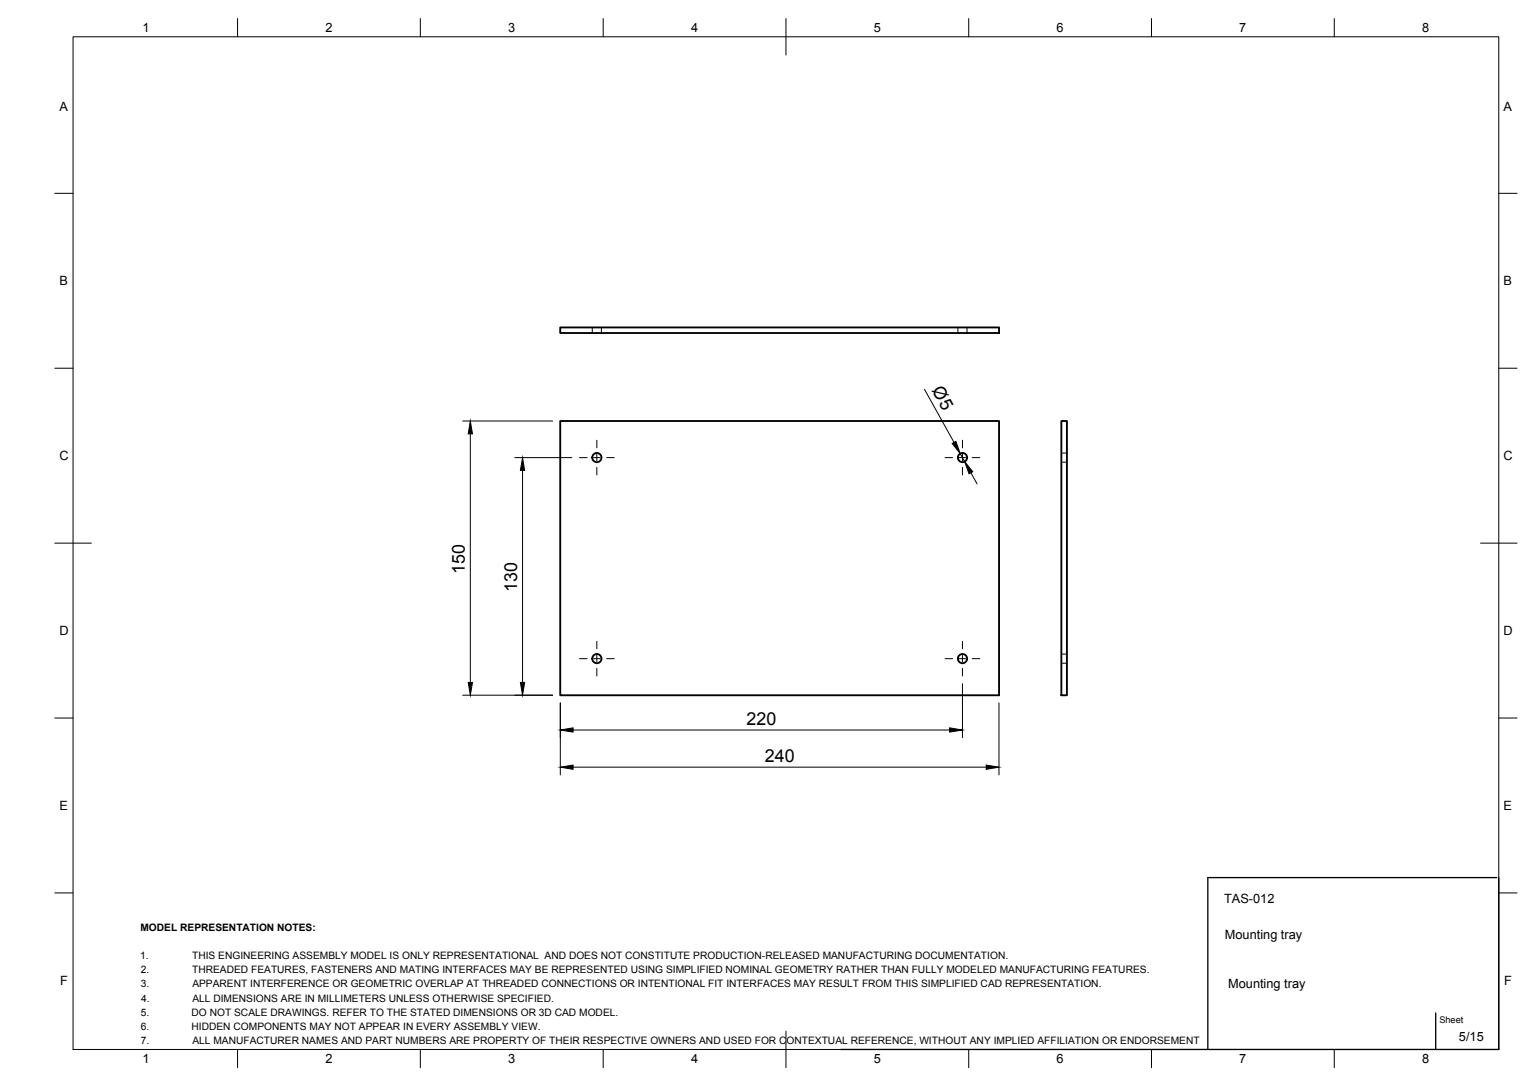
ISO-10303-21;
HEADER;
/* Generated by software containing ST-Developer
 * from STEP Tools, Inc. (www.steptools.com) 
 */

FILE_DESCRIPTION(
/* description */ (
'Independent welded steel electronics enclosure with removable sealed 
lid, internal mounting tray and two threaded cable entries. 300 x 220 
mm body. No ingress or electrical safety rating assigned.'),
/* implementation_level */ '2;1');

FILE_NAME(
/* name */ 'Mounting tray.step',
/* time_stamp */ '2026-11-14T09:13:27-08:00',
/* author */ (''),
/* organization */ (''),
/* preprocessor_version */ 'ST-DEVELOPER v20.2',
/* originating_system */ 'Autodesk Translation Framework v15.17.0.0',
/* authorisation */ '');

FILE_SCHEMA (('AUTOMOTIVE_DESIGN { 1 0 10303 214 3 1 1 }'));
ENDSEC;

DATA;
#10=MECHANICAL_DESIGN_GEOMETRIC_PRESENTATION_REPRESENTATION('',(#975),#94412);
#945=SHAPE_REPRESENTATION_RELATIONSHIP('SRR','None',#94497,#960);
#960=ADVANCED_BREP_SHAPE_REPRESENTATION('',(#990),#94406);
#975=STYLED_ITEM('',(#94580),#990);
#990=MANIFOLD_SOLID_BREP('Body1',#8260);
#1035=FACE_BOUND('',#1790,.T.);
#1036=FACE_BOUND('',#1791,.T.);
#1037=FACE_BOUND('',#1792,.T.);
#1038=FACE_BOUND('',#1793,.T.);
#1039=FACE_BOUND('',#1795,.T.);
#1040=FACE_BOUND('',#1796,.T.);
#1041=FACE_BOUND('',#1797,.T.);
#1042=FACE_BOUND('',#1798,.T.);
#1125=PLANE('',#8767);
#1126=PLANE('',#8768);
#1127=PLANE('',#8769);
#1128=PLANE('',#8770);
#1129=PLANE('',#8771);
#1130=PLANE('',#8772);
#1386=FACE_OUTER_BOUND('',#1781,.T.);
#1387=FACE_OUTER_BOUND('',#1782,.T.);
#1388=FACE_OUTER_BOUND('',#1783,.T.);
#1389=FACE_OUTER_BOUND('',#1784,.T.);
#1390=FACE_OUTER_BOUND('',#1785,.T.);
#1391=FACE_OUTER_BOUND('',#1786,.T.);
#1392=FACE_OUTER_BOUND('',#1787,.T.);
#1393=FACE_OUTER_BOUND('',#1788,.T.);
#1394=FACE_OUTER_BOUND('',#1789,.T.);
#1395=FACE_OUTER_BOUND('',#1794,.T.);
#1781=EDGE_LOOP('',(#6764,#6765,#6766,#6767));
#1782=EDGE_LOOP('',(#6768,#6769,#6770,#6771));
#1783=EDGE_LOOP('',(#6772,#6773,#6774,#6775));
#1784=EDGE_LOOP('',(#6776,#6777,#6778,#6779));
#1785=EDGE_LOOP('',(#6780,#6781,#6782,#6783));
#1786=EDGE_LOOP('',(#6784,#6785,#6786,#6787));
#1787=EDGE_LOOP('',(#6788,#6789,#6790,#6791));
#1788=EDGE_LOOP('',(#6792,#6793,#6794,#6795));
#1789=EDGE_LOOP('',(#6796,#6797,#6798,#6799));
#1790=EDGE_LOOP('',(#6800));
#1791=EDGE_LOOP('',(#6801));
#1792=EDGE_LOOP('',(#6802));
#1793=EDGE_LOOP('',(#6803));
#1794=EDGE_LOOP('',(#6804,#6805,#6806,#6807));
#1795=EDGE_LOOP('',(#6808));
#1796=EDGE_LOOP('',(#6809));
#1797=EDGE_LOOP('',(#6810));
#1798=EDGE_LOOP('',(#6811));
#2203=LINE('',#59828,#2601);
#2204=LINE('',#59834,#2602);
#2205=LINE('',#59840,#2603);
#2206=LINE('',#59846,#2604);
#2207=LINE('',#59851,#2605);
#2208=LINE('',#59853,#2606);
#2209=LINE('',#59855,#2607);
#2210=LINE('',#59856,#2608);
#2211=LINE('',#59859,#2609);
#2212=LINE('',#59861,#2610);
#2213=LINE('',#59862,#2611);
#2214=LINE('',#59865,#2612);
#2215=LINE('',#59867,#2613);
#2216=LINE('',#59868,#2614);
#2217=LINE('',#59870,#2615);
#2218=LINE('',#59871,#2616);
#2601=VECTOR('',#9863,2.5);
#2602=VECTOR('',#9870,2.5);
#2603=VECTOR('',#9877,2.5);
#2604=VECTOR('',#9884,2.5);
#2605=VECTOR('',#9889,10.);
#2606=VECTOR('',#9890,10.);
#2607=VECTOR('',#9891,10.);
#2608=VECTOR('',#9892,10.);
#2609=VECTOR('',#9895,10.);
#2610=VECTOR('',#9896,10.);
#2611=VECTOR('',#9897,10.);
#2612=VECTOR('',#9900,10.);
#2613=VECTOR('',#9901,10.);
#2614=VECTOR('',#9902,10.);
#2615=VECTOR('',#9905,10.);
#2616=VECTOR('',#9906,10.);
#2802=CIRCLE('',#8756,2.5);
#2803=CIRCLE('',#8757,2.5);
#2804=CIRCLE('',#8759,2.5);
#2805=CIRCLE('',#8760,2.5);
#2806=CIRCLE('',#8762,2.5);
#2807=CIRCLE('',#8763,2.5);
#2808=CIRCLE('',#8765,2.5);
#2809=CIRCLE('',#8766,2.5);
#3476=VERTEX_POINT('',#59825);
#3477=VERTEX_POINT('',#59827);
#3478=VERTEX_POINT('',#59831);
#3479=VERTEX_POINT('',#59833);
#3480=VERTEX_POINT('',#59837);
#3481=VERTEX_POINT('',#59839);
#3482=VERTEX_POINT('',#59843);
#3483=VERTEX_POINT('',#59845);
#3484=VERTEX_POINT('',#59849);
#3485=VERTEX_POINT('',#59850);
#3486=VERTEX_POINT('',#59852);
#3487=VERTEX_POINT('',#59854);
#3488=VERTEX_POINT('',#59858);
#3489=VERTEX_POINT('',#59860);
#3490=VERTEX_POINT('',#59864);
#3491=VERTEX_POINT('',#59866);
#4647=EDGE_CURVE('',#3476,#3476,#2802,.T.);
#4648=EDGE_CURVE('',#3476,#3477,#2203,.T.);
#4649=EDGE_CURVE('',#3477,#3477,#2803,.T.);
#4650=EDGE_CURVE('',#3478,#3478,#2804,.T.);
#4651=EDGE_CURVE('',#3478,#3479,#2204,.T.);
#4652=EDGE_CURVE('',#3479,#3479,#2805,.T.);
#4653=EDGE_CURVE('',#3480,#3480,#2806,.T.);
#4654=EDGE_CURVE('',#3480,#3481,#2205,.T.);
#4655=EDGE_CURVE('',#3481,#3481,#2807,.T.);
#4656=EDGE_CURVE('',#3482,#3482,#2808,.T.);
#4657=EDGE_CURVE('',#3482,#3483,#2206,.T.);
#4658=EDGE_CURVE('',#3483,#3483,#2809,.T.);
#4659=EDGE_CURVE('',#3484,#3485,#2207,.T.);
#4660=EDGE_CURVE('',#3485,#3486,#2208,.T.);
#4661=EDGE_CURVE('',#3487,#3486,#2209,.T.);
#4662=EDGE_CURVE('',#3484,#3487,#2210,.T.);
#4663=EDGE_CURVE('',#3488,#3484,#2211,.T.);
#4664=EDGE_CURVE('',#3489,#3487,#2212,.T.);
#4665=EDGE_CURVE('',#3488,#3489,#2213,.T.);
#4666=EDGE_CURVE('',#3490,#3488,#2214,.T.);
#4667=EDGE_CURVE('',#3491,#3489,#2215,.T.);
#4668=EDGE_CURVE('',#3490,#3491,#2216,.T.);
#4669=EDGE_CURVE('',#3485,#3490,#2217,.T.);
#4670=EDGE_CURVE('',#3486,#3491,#2218,.T.);
#6764=ORIENTED_EDGE('',*,*,#4647,.F.);
#6765=ORIENTED_EDGE('',*,*,#4648,.T.);
#6766=ORIENTED_EDGE('',*,*,#4649,.F.);
#6767=ORIENTED_EDGE('',*,*,#4648,.F.);
#6768=ORIENTED_EDGE('',*,*,#4650,.F.);
#6769=ORIENTED_EDGE('',*,*,#4651,.T.);
#6770=ORIENTED_EDGE('',*,*,#4652,.F.);
#6771=ORIENTED_EDGE('',*,*,#4651,.F.);
#6772=ORIENTED_EDGE('',*,*,#4653,.F.);
#6773=ORIENTED_EDGE('',*,*,#4654,.T.);
#6774=ORIENTED_EDGE('',*,*,#4655,.F.);
#6775=ORIENTED_EDGE('',*,*,#4654,.F.);
#6776=ORIENTED_EDGE('',*,*,#4656,.F.);
#6777=ORIENTED_EDGE('',*,*,#4657,.T.);
#6778=ORIENTED_EDGE('',*,*,#4658,.F.);
#6779=ORIENTED_EDGE('',*,*,#4657,.F.);
#6780=ORIENTED_EDGE('',*,*,#4659,.T.);
#6781=ORIENTED_EDGE('',*,*,#4660,.T.);
#6782=ORIENTED_EDGE('',*,*,#4661,.F.);
#6783=ORIENTED_EDGE('',*,*,#4662,.F.);
#6784=ORIENTED_EDGE('',*,*,#4663,.T.);
#6785=ORIENTED_EDGE('',*,*,#4662,.T.);
#6786=ORIENTED_EDGE('',*,*,#4664,.F.);
#6787=ORIENTED_EDGE('',*,*,#4665,.F.);
#6788=ORIENTED_EDGE('',*,*,#4666,.T.);
#6789=ORIENTED_EDGE('',*,*,#4665,.T.);
#6790=ORIENTED_EDGE('',*,*,#4667,.F.);
#6791=ORIENTED_EDGE('',*,*,#4668,.F.);
#6792=ORIENTED_EDGE('',*,*,#4669,.T.);
#6793=ORIENTED_EDGE('',*,*,#4668,.T.);
#6794=ORIENTED_EDGE('',*,*,#4670,.F.);
#6795=ORIENTED_EDGE('',*,*,#4660,.F.);
#6796=ORIENTED_EDGE('',*,*,#4670,.T.);
#6797=ORIENTED_EDGE('',*,*,#4667,.T.);
#6798=ORIENTED_EDGE('',*,*,#4664,.T.);
#6799=ORIENTED_EDGE('',*,*,#4661,.T.);
#6800=ORIENTED_EDGE('',*,*,#4647,.T.);
#6801=ORIENTED_EDGE('',*,*,#4650,.T.);
#6802=ORIENTED_EDGE('',*,*,#4653,.T.);
#6803=ORIENTED_EDGE('',*,*,#4656,.T.);
#6804=ORIENTED_EDGE('',*,*,#4669,.F.);
#6805=ORIENTED_EDGE('',*,*,#4659,.F.);
#6806=ORIENTED_EDGE('',*,*,#4663,.F.);
#6807=ORIENTED_EDGE('',*,*,#4666,.F.);
#6808=ORIENTED_EDGE('',*,*,#4649,.T.);
#6809=ORIENTED_EDGE('',*,*,#4652,.T.);
#6810=ORIENTED_EDGE('',*,*,#4655,.T.);
#6811=ORIENTED_EDGE('',*,*,#4658,.T.);
#7810=CYLINDRICAL_SURFACE('',#8755,2.5);
#7811=CYLINDRICAL_SURFACE('',#8758,2.5);
#7812=CYLINDRICAL_SURFACE('',#8761,2.5);
#7813=CYLINDRICAL_SURFACE('',#8764,2.5);
#8123=ADVANCED_FACE('',(#1386),#7810,.F.);
#8124=ADVANCED_FACE('',(#1387),#7811,.F.);
#8125=ADVANCED_FACE('',(#1388),#7812,.F.);
#8126=ADVANCED_FACE('',(#1389),#7813,.F.);
#8127=ADVANCED_FACE('',(#1390),#1125,.T.);
#8128=ADVANCED_FACE('',(#1391),#1126,.T.);
#8129=ADVANCED_FACE('',(#1392),#1127,.T.);
#8130=ADVANCED_FACE('',(#1393),#1128,.T.);
#8131=ADVANCED_FACE('',(#1394,#1035,#1036,#1037,#1038),#1129,.T.);
#8132=ADVANCED_FACE('',(#1395,#1039,#1040,#1041,#1042),#1130,.F.);
#8260=CLOSED_SHELL('',(#8123,#8124,#8125,#8126,#8127,#8128,#8129,#8130,
#8131,#8132));
#8754=AXIS2_PLACEMENT_3D('',#59823,#9857,#9858);
#8755=AXIS2_PLACEMENT_3D('',#59824,#9859,#9860);
#8756=AXIS2_PLACEMENT_3D('',#59826,#9861,#9862);
#8757=AXIS2_PLACEMENT_3D('',#59829,#9864,#9865);
#8758=AXIS2_PLACEMENT_3D('',#59830,#9866,#9867);
#8759=AXIS2_PLACEMENT_3D('',#59832,#9868,#9869);
#8760=AXIS2_PLACEMENT_3D('',#59835,#9871,#9872);
#8761=AXIS2_PLACEMENT_3D('',#59836,#9873,#9874);
#8762=AXIS2_PLACEMENT_3D('',#59838,#9875,#9876);
#8763=AXIS2_PLACEMENT_3D('',#59841,#9878,#9879);
#8764=AXIS2_PLACEMENT_3D('',#59842,#9880,#9881);
#8765=AXIS2_PLACEMENT_3D('',#59844,#9882,#9883);
#8766=AXIS2_PLACEMENT_3D('',#59847,#9885,#9886);
#8767=AXIS2_PLACEMENT_3D('',#59848,#9887,#9888);
#8768=AXIS2_PLACEMENT_3D('',#59857,#9893,#9894);
#8769=AXIS2_PLACEMENT_3D('',#59863,#9898,#9899);
#8770=AXIS2_PLACEMENT_3D('',#59869,#9903,#9904);
#8771=AXIS2_PLACEMENT_3D('',#59872,#9907,#9908);
#8772=AXIS2_PLACEMENT_3D('',#59873,#9909,#9910);
#9857=DIRECTION('axis',(0.,0.,1.));
#9858=DIRECTION('refdir',(1.,0.,0.));
#9859=DIRECTION('center_axis',(0.,0.,-1.));
#9860=DIRECTION('ref_axis',(1.,0.,0.));
#9861=DIRECTION('center_axis',(0.,0.,-1.));
#9862=DIRECTION('ref_axis',(1.,0.,0.));
#9863=DIRECTION('',(0.,0.,-1.));
#9864=DIRECTION('center_axis',(0.,0.,1.));
#9865=DIRECTION('ref_axis',(1.,0.,0.));
#9866=DIRECTION('center_axis',(0.,0.,-1.));
#9867=DIRECTION('ref_axis',(1.,0.,0.));
#9868=DIRECTION('center_axis',(0.,0.,-1.));
#9869=DIRECTION('ref_axis',(1.,0.,0.));
#9870=DIRECTION('',(0.,0.,-1.));
#9871=DIRECTION('center_axis',(0.,0.,1.));
#9872=DIRECTION('ref_axis',(1.,0.,0.));
#9873=DIRECTION('center_axis',(0.,0.,-1.));
#9874=DIRECTION('ref_axis',(1.,0.,0.));
#9875=DIRECTION('center_axis',(0.,0.,-1.));
#9876=DIRECTION('ref_axis',(1.,0.,0.));
#9877=DIRECTION('',(0.,0.,-1.));
#9878=DIRECTION('center_axis',(0.,0.,1.));
#9879=DIRECTION('ref_axis',(1.,0.,0.));
#9880=DIRECTION('center_axis',(0.,0.,-1.));
#9881=DIRECTION('ref_axis',(1.,0.,0.));
#9882=DIRECTION('center_axis',(0.,0.,-1.));
#9883=DIRECTION('ref_axis',(1.,0.,0.));
#9884=DIRECTION('',(0.,0.,-1.));
#9885=DIRECTION('center_axis',(0.,0.,1.));
#9886=DIRECTION('ref_axis',(1.,0.,0.));
#9887=DIRECTION('center_axis',(0.,1.,0.));
#9888=DIRECTION('ref_axis',(-1.,0.,0.));
#9889=DIRECTION('',(-1.,0.,0.));
#9890=DIRECTION('',(0.,0.,1.));
#9891=DIRECTION('',(-1.,0.,0.));
#9892=DIRECTION('',(0.,0.,1.));
#9893=DIRECTION('center_axis',(1.,0.,0.));
#9894=DIRECTION('ref_axis',(0.,1.,0.));
#9895=DIRECTION('',(0.,1.,0.));
#9896=DIRECTION('',(0.,1.,0.));
#9897=DIRECTION('',(0.,0.,1.));
#9898=DIRECTION('center_axis',(0.,-1.,0.));
#9899=DIRECTION('ref_axis',(1.,0.,0.));
#9900=DIRECTION('',(1.,0.,0.));
#9901=DIRECTION('',(1.,0.,0.));
#9902=DIRECTION('',(0.,0.,1.));
#9903=DIRECTION('center_axis',(-1.,0.,0.));
#9904=DIRECTION('ref_axis',(0.,-1.,0.));
#9905=DIRECTION('',(0.,-1.,0.));
#9906=DIRECTION('',(0.,-1.,0.));
#9907=DIRECTION('center_axis',(0.,0.,1.));
#9908=DIRECTION('ref_axis',(1.,0.,0.));
#9909=DIRECTION('center_axis',(0.,0.,1.));
#9910=DIRECTION('ref_axis',(1.,0.,0.));
#59823=CARTESIAN_POINT('',(0.,0.,0.));
#59824=CARTESIAN_POINT('Origin',(100.,-55.,1.5));
#59825=CARTESIAN_POINT('',(97.5,-55.,3.));
#59826=CARTESIAN_POINT('Origin',(100.,-55.,3.));
#59827=CARTESIAN_POINT('',(97.5,-55.,0.));
#59828=CARTESIAN_POINT('',(97.5,-55.,1.5));
#59829=CARTESIAN_POINT('Origin',(100.,-55.,0.));
#59830=CARTESIAN_POINT('Origin',(-100.,-55.,1.5));
#59831=CARTESIAN_POINT('',(-102.5,-55.,3.));
#59832=CARTESIAN_POINT('Origin',(-100.,-55.,3.));
#59833=CARTESIAN_POINT('',(-102.5,-55.,0.));
#59834=CARTESIAN_POINT('',(-102.5,-55.,1.5));
#59835=CARTESIAN_POINT('Origin',(-100.,-55.,0.));
#59836=CARTESIAN_POINT('Origin',(-100.,55.,1.5));
#59837=CARTESIAN_POINT('',(-102.5,55.,3.));
#59838=CARTESIAN_POINT('Origin',(-100.,55.,3.));
#59839=CARTESIAN_POINT('',(-102.5,55.,0.));
#59840=CARTESIAN_POINT('',(-102.5,55.,1.5));
#59841=CARTESIAN_POINT('Origin',(-100.,55.,0.));
#59842=CARTESIAN_POINT('Origin',(100.,55.,1.5));
#59843=CARTESIAN_POINT('',(97.5,55.,3.));
#59844=CARTESIAN_POINT('Origin',(100.,55.,3.));
#59845=CARTESIAN_POINT('',(97.5,55.,0.));
#59846=CARTESIAN_POINT('',(97.5,55.,1.5));
#59847=CARTESIAN_POINT('Origin',(100.,55.,0.));
#59848=CARTESIAN_POINT('Origin',(120.,75.,0.));
#59849=CARTESIAN_POINT('',(120.,75.,0.));
#59850=CARTESIAN_POINT('',(-120.,75.,0.));
#59851=CARTESIAN_POINT('',(120.,75.,0.));
#59852=CARTESIAN_POINT('',(-120.,75.,3.));
#59853=CARTESIAN_POINT('',(-120.,75.,0.));
#59854=CARTESIAN_POINT('',(120.,75.,3.));
#59855=CARTESIAN_POINT('',(120.,75.,3.));
#59856=CARTESIAN_POINT('',(120.,75.,0.));
#59857=CARTESIAN_POINT('Origin',(120.,-75.,0.));
#59858=CARTESIAN_POINT('',(120.,-75.,0.));
#59859=CARTESIAN_POINT('',(120.,-75.,0.));
#59860=CARTESIAN_POINT('',(120.,-75.,3.));
#59861=CARTESIAN_POINT('',(120.,-75.,3.));
#59862=CARTESIAN_POINT('',(120.,-75.,0.));
#59863=CARTESIAN_POINT('Origin',(-120.,-75.,0.));
#59864=CARTESIAN_POINT('',(-120.,-75.,0.));
#59865=CARTESIAN_POINT('',(-120.,-75.,0.));
#59866=CARTESIAN_POINT('',(-120.,-75.,3.));
#59867=CARTESIAN_POINT('',(-120.,-75.,3.));
#59868=CARTESIAN_POINT('',(-120.,-75.,0.));
#59869=CARTESIAN_POINT('Origin',(-120.,75.,0.));
#59870=CARTESIAN_POINT('',(-120.,75.,0.));
#59871=CARTESIAN_POINT('',(-120.,75.,3.));
#59872=CARTESIAN_POINT('Origin',(0.,0.,3.));
#59873=CARTESIAN_POINT('Origin',(0.,0.,0.));
#94388=UNCERTAINTY_MEASURE_WITH_UNIT(LENGTH_MEASURE(0.01),#94413,
'DISTANCE_ACCURACY_VALUE',
'Maximum model space distance between geometric entities at asserted c
onnectivities');
#94394=UNCERTAINTY_MEASURE_WITH_UNIT(LENGTH_MEASURE(0.01),#94413,
'DISTANCE_ACCURACY_VALUE',
'Maximum model space distance between geometric entities at asserted c
onnectivities');
#94406=(
GEOMETRIC_REPRESENTATION_CONTEXT(3)
GLOBAL_UNCERTAINTY_ASSIGNED_CONTEXT((#94388))
GLOBAL_UNIT_ASSIGNED_CONTEXT((#94413,#94415,#94416))
REPRESENTATION_CONTEXT('','3D')
);
#94412=(
GEOMETRIC_REPRESENTATION_CONTEXT(3)
GLOBAL_UNCERTAINTY_ASSIGNED_CONTEXT((#94394))
GLOBAL_UNIT_ASSIGNED_CONTEXT((#94413,#94415,#94416))
REPRESENTATION_CONTEXT('','3D')
);
#94413=(
LENGTH_UNIT()
NAMED_UNIT(*)
SI_UNIT(.MILLI.,.METRE.)
);
#94415=(
NAMED_UNIT(*)
PLANE_ANGLE_UNIT()
SI_UNIT($,.RADIAN.)
);
#94416=(
NAMED_UNIT(*)
SI_UNIT($,.STERADIAN.)
SOLID_ANGLE_UNIT()
);
#94428=SHAPE_DEFINITION_REPRESENTATION(#94462,#94497);
#94462=PRODUCT_DEFINITION_SHAPE('',$,#94515);
#94497=SHAPE_REPRESENTATION('',(#8754),#94406);
#94503=PRODUCT_DEFINITION_CONTEXT('part definition',#94556,'design');
#94515=PRODUCT_DEFINITION('Mounting tray','Mounting tray',#94532,#94503);
#94532=PRODUCT_DEFINITION_FORMATION('',$,#94569);
#94556=APPLICATION_CONTEXT(
'Core Data for Automotive Mechanical Design Process');
#94557=PRODUCT_CONTEXT('part definition',#94556,'mechanical');
#94569=PRODUCT('Mounting tray','Mounting tray',$,(#94557));
#94580=PRESENTATION_STYLE_ASSIGNMENT((#94587));
#94587=SURFACE_STYLE_USAGE(.BOTH.,#94594);
#94594=SURFACE_SIDE_STYLE('',(#94601));
#94601=SURFACE_STYLE_FILL_AREA(#94608);
#94608=FILL_AREA_STYLE('Opaque(81,175,227)',(#94615));
#94615=FILL_AREA_STYLE_COLOUR('Opaque(81,175,227)',#94622);
#94622=COLOUR_RGB('Opaque(81,175,227)',0.317647058823529,0.686274509803922,
0.890196078431372);
ENDSEC;
END-ISO-10303-21;
